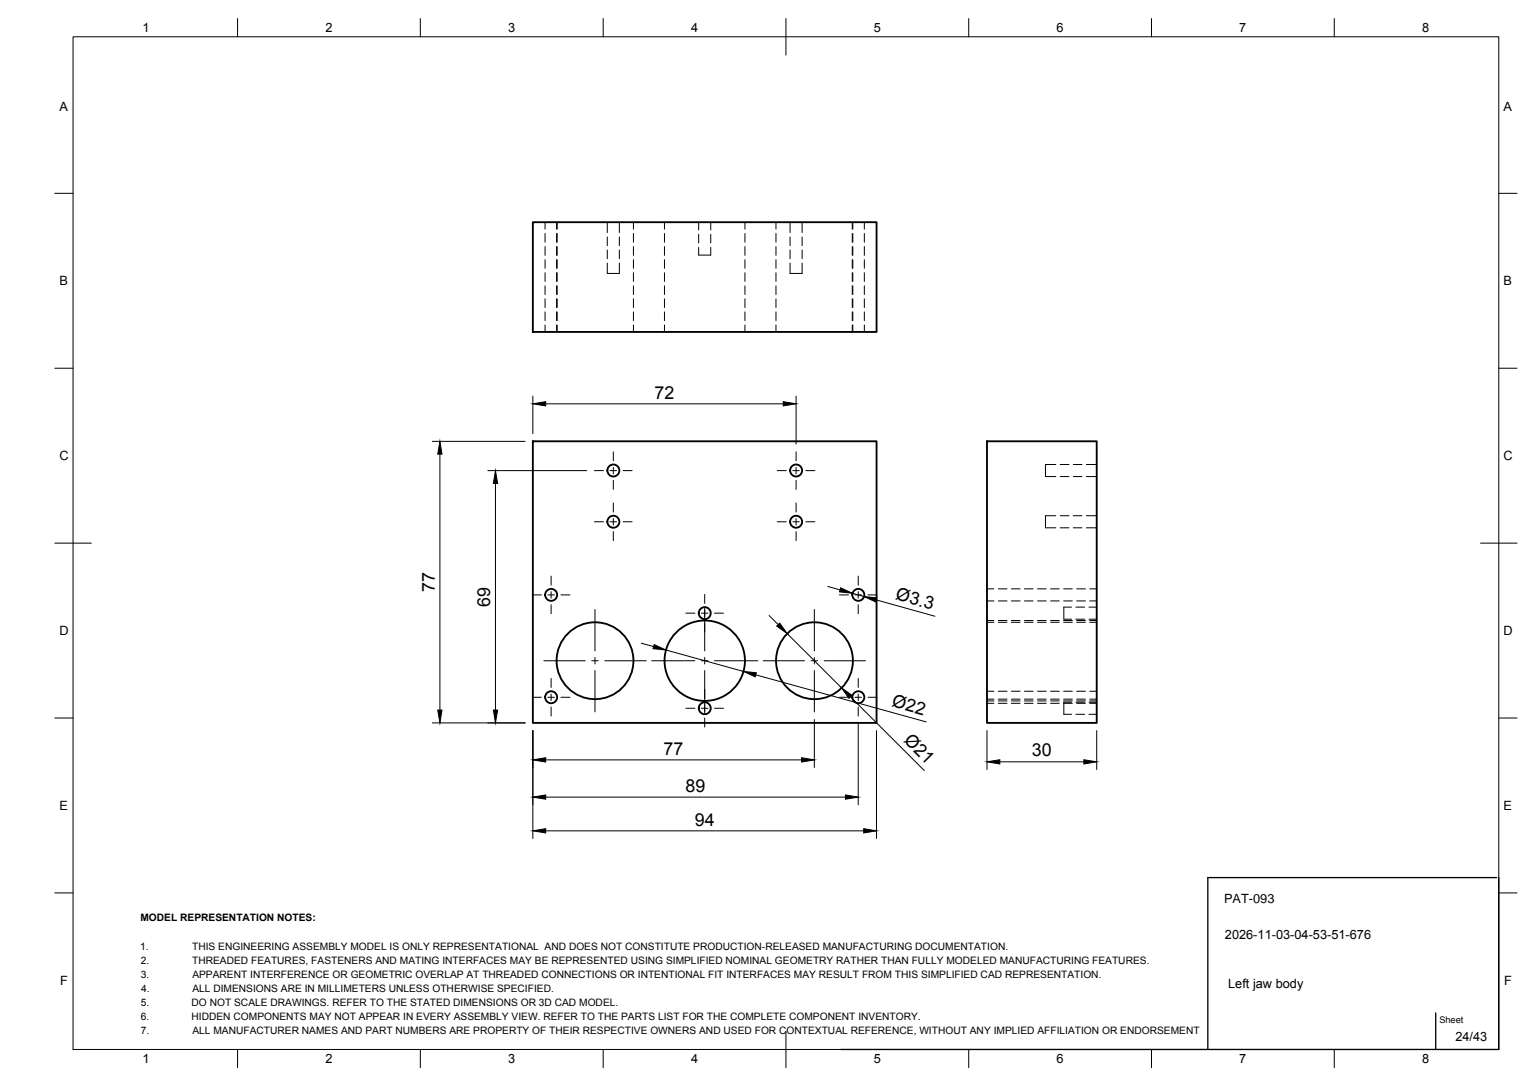
ISO-10303-21;
HEADER;
/* Generated by software containing ST-Developer
 * from STEP Tools, Inc. (www.steptools.com) 
 */

FILE_DESCRIPTION(
/* description */ ('Self-centering screw clamp'),
/* implementation_level */ '2;1');

FILE_NAME(
/* name */ 'Left jaw body.step',
/* time_stamp */ '2026-10-28T03:25:31-07:00',
/* author */ (''),
/* organization */ (''),
/* preprocessor_version */ 'ST-DEVELOPER v20.2',
/* originating_system */ 'Autodesk Translation Framework v15.17.0.0',
/* authorisation */ '');

FILE_SCHEMA (('AUTOMOTIVE_DESIGN { 1 0 10303 214 3 1 1 }'));
ENDSEC;

DATA;
#10=MECHANICAL_DESIGN_GEOMETRIC_PRESENTATION_REPRESENTATION('',(#650),#16799);
#561=SHAPE_REPRESENTATION_RELATIONSHIP('SRR','None',#17036,#602);
#602=ADVANCED_BREP_SHAPE_REPRESENTATION('',(#698),#16774);
#650=STYLED_ITEM('',(#17305),#698);
#698=MANIFOLD_SOLID_BREP('Body1',#9101);
#851=FACE_BOUND('',#2160,.T.);
#852=FACE_BOUND('',#2161,.T.);
#853=FACE_BOUND('',#2162,.T.);
#854=FACE_BOUND('',#2163,.T.);
#855=FACE_BOUND('',#2164,.T.);
#856=FACE_BOUND('',#2165,.T.);
#857=FACE_BOUND('',#2166,.T.);
#858=FACE_BOUND('',#2167,.T.);
#859=FACE_BOUND('',#2168,.T.);
#860=FACE_BOUND('',#2169,.T.);
#861=FACE_BOUND('',#2170,.T.);
#862=FACE_BOUND('',#2171,.T.);
#863=FACE_BOUND('',#2172,.T.);
#864=FACE_BOUND('',#2175,.T.);
#865=FACE_BOUND('',#2176,.T.);
#866=FACE_BOUND('',#2177,.T.);
#867=FACE_BOUND('',#2178,.T.);
#868=FACE_BOUND('',#2179,.T.);
#869=FACE_BOUND('',#2180,.T.);
#870=FACE_BOUND('',#2181,.T.);
#1122=PLANE('',#10087);
#1123=PLANE('',#10091);
#1124=PLANE('',#10095);
#1125=PLANE('',#10099);
#1126=PLANE('',#10103);
#1127=PLANE('',#10107);
#1128=PLANE('',#10129);
#1129=PLANE('',#10130);
#1130=PLANE('',#10131);
#1131=PLANE('',#10132);
#1132=PLANE('',#10133);
#1133=PLANE('',#10134);
#1502=FACE_OUTER_BOUND('',#2139,.T.);
#1503=FACE_OUTER_BOUND('',#2140,.T.);
#1504=FACE_OUTER_BOUND('',#2141,.T.);
#1505=FACE_OUTER_BOUND('',#2142,.T.);
#1506=FACE_OUTER_BOUND('',#2143,.T.);
#1507=FACE_OUTER_BOUND('',#2144,.T.);
#1508=FACE_OUTER_BOUND('',#2145,.T.);
#1509=FACE_OUTER_BOUND('',#2146,.T.);
#1510=FACE_OUTER_BOUND('',#2147,.T.);
#1511=FACE_OUTER_BOUND('',#2148,.T.);
#1512=FACE_OUTER_BOUND('',#2149,.T.);
#1513=FACE_OUTER_BOUND('',#2150,.T.);
#1514=FACE_OUTER_BOUND('',#2151,.T.);
#1515=FACE_OUTER_BOUND('',#2152,.T.);
#1516=FACE_OUTER_BOUND('',#2153,.T.);
#1517=FACE_OUTER_BOUND('',#2154,.T.);
#1518=FACE_OUTER_BOUND('',#2155,.T.);
#1519=FACE_OUTER_BOUND('',#2156,.T.);
#1520=FACE_OUTER_BOUND('',#2157,.T.);
#1521=FACE_OUTER_BOUND('',#2158,.T.);
#1522=FACE_OUTER_BOUND('',#2159,.T.);
#1523=FACE_OUTER_BOUND('',#2173,.T.);
#1524=FACE_OUTER_BOUND('',#2174,.T.);
#1525=FACE_OUTER_BOUND('',#2182,.T.);
#1526=FACE_OUTER_BOUND('',#2183,.T.);
#2139=EDGE_LOOP('',(#7191,#7192,#7193,#7194));
#2140=EDGE_LOOP('',(#7195));
#2141=EDGE_LOOP('',(#7196,#7197,#7198,#7199));
#2142=EDGE_LOOP('',(#7200));
#2143=EDGE_LOOP('',(#7201,#7202,#7203,#7204));
#2144=EDGE_LOOP('',(#7205));
#2145=EDGE_LOOP('',(#7206,#7207,#7208,#7209));
#2146=EDGE_LOOP('',(#7210));
#2147=EDGE_LOOP('',(#7211,#7212,#7213,#7214));
#2148=EDGE_LOOP('',(#7215));
#2149=EDGE_LOOP('',(#7216,#7217,#7218,#7219));
#2150=EDGE_LOOP('',(#7220));
#2151=EDGE_LOOP('',(#7221,#7222,#7223,#7224));
#2152=EDGE_LOOP('',(#7225,#7226,#7227,#7228));
#2153=EDGE_LOOP('',(#7229,#7230,#7231,#7232));
#2154=EDGE_LOOP('',(#7233,#7234,#7235,#7236));
#2155=EDGE_LOOP('',(#7237,#7238,#7239,#7240));
#2156=EDGE_LOOP('',(#7241,#7242,#7243,#7244));
#2157=EDGE_LOOP('',(#7245,#7246,#7247,#7248));
#2158=EDGE_LOOP('',(#7249,#7250,#7251,#7252));
#2159=EDGE_LOOP('',(#7253,#7254,#7255,#7256));
#2160=EDGE_LOOP('',(#7257));
#2161=EDGE_LOOP('',(#7258));
#2162=EDGE_LOOP('',(#7259));
#2163=EDGE_LOOP('',(#7260));
#2164=EDGE_LOOP('',(#7261));
#2165=EDGE_LOOP('',(#7262));
#2166=EDGE_LOOP('',(#7263));
#2167=EDGE_LOOP('',(#7264));
#2168=EDGE_LOOP('',(#7265));
#2169=EDGE_LOOP('',(#7266));
#2170=EDGE_LOOP('',(#7267));
#2171=EDGE_LOOP('',(#7268));
#2172=EDGE_LOOP('',(#7269));
#2173=EDGE_LOOP('',(#7270,#7271,#7272,#7273));
#2174=EDGE_LOOP('',(#7274,#7275,#7276,#7277));
#2175=EDGE_LOOP('',(#7278));
#2176=EDGE_LOOP('',(#7279));
#2177=EDGE_LOOP('',(#7280));
#2178=EDGE_LOOP('',(#7281));
#2179=EDGE_LOOP('',(#7282));
#2180=EDGE_LOOP('',(#7283));
#2181=EDGE_LOOP('',(#7284));
#2182=EDGE_LOOP('',(#7285,#7286,#7287,#7288));
#2183=EDGE_LOOP('',(#7289,#7290,#7291,#7292));
#2842=LINE('',#15213,#3415);
#2843=LINE('',#15220,#3416);
#2844=LINE('',#15227,#3417);
#2845=LINE('',#15234,#3418);
#2846=LINE('',#15241,#3419);
#2847=LINE('',#15248,#3420);
#2848=LINE('',#15255,#3421);
#2849=LINE('',#15261,#3422);
#2850=LINE('',#15267,#3423);
#2851=LINE('',#15273,#3424);
#2852=LINE('',#15279,#3425);
#2853=LINE('',#15285,#3426);
#2854=LINE('',#15291,#3427);
#2855=LINE('',#15296,#3428);
#2856=LINE('',#15298,#3429);
#2857=LINE('',#15300,#3430);
#2858=LINE('',#15301,#3431);
#2859=LINE('',#15304,#3432);
#2860=LINE('',#15306,#3433);
#2861=LINE('',#15307,#3434);
#2862=LINE('',#15310,#3435);
#2863=LINE('',#15312,#3436);
#2864=LINE('',#15313,#3437);
#2865=LINE('',#15315,#3438);
#2866=LINE('',#15316,#3439);
#3415=VECTOR('',#12035,0.165);
#3416=VECTOR('',#12044,0.164999999999999);
#3417=VECTOR('',#12053,0.165);
#3418=VECTOR('',#12062,0.164999999999999);
#3419=VECTOR('',#12071,0.165);
#3420=VECTOR('',#12080,0.165);
#3421=VECTOR('',#12089,0.165);
#3422=VECTOR('',#12096,0.165);
#3423=VECTOR('',#12103,0.165);
#3424=VECTOR('',#12110,0.165);
#3425=VECTOR('',#12117,1.1);
#3426=VECTOR('',#12124,1.05);
#3427=VECTOR('',#12131,1.05);
#3428=VECTOR('',#12136,1.);
#3429=VECTOR('',#12137,1.);
#3430=VECTOR('',#12138,1.);
#3431=VECTOR('',#12139,1.);
#3432=VECTOR('',#12142,1.);
#3433=VECTOR('',#12143,1.);
#3434=VECTOR('',#12144,1.);
#3435=VECTOR('',#12147,1.);
#3436=VECTOR('',#12148,1.);
#3437=VECTOR('',#12149,1.);
#3438=VECTOR('',#12152,1.);
#3439=VECTOR('',#12153,1.);
#3972=CIRCLE('',#10085,0.165);
#3973=CIRCLE('',#10086,0.165);
#3974=CIRCLE('',#10089,0.164999999999999);
#3975=CIRCLE('',#10090,0.164999999999999);
#3976=CIRCLE('',#10093,0.165);
#3977=CIRCLE('',#10094,0.165);
#3978=CIRCLE('',#10097,0.164999999999999);
#3979=CIRCLE('',#10098,0.164999999999999);
#3980=CIRCLE('',#10101,0.165);
#3981=CIRCLE('',#10102,0.165);
#3982=CIRCLE('',#10105,0.165);
#3983=CIRCLE('',#10106,0.165);
#3984=CIRCLE('',#10109,0.165);
#3985=CIRCLE('',#10110,0.165);
#3986=CIRCLE('',#10112,0.165);
#3987=CIRCLE('',#10113,0.165);
#3988=CIRCLE('',#10115,0.165);
#3989=CIRCLE('',#10116,0.165);
#3990=CIRCLE('',#10118,0.165);
#3991=CIRCLE('',#10119,0.165);
#3992=CIRCLE('',#10121,1.1);
#3993=CIRCLE('',#10122,1.1);
#3994=CIRCLE('',#10124,1.05);
#3995=CIRCLE('',#10125,1.05);
#3996=CIRCLE('',#10127,1.05);
#3997=CIRCLE('',#10128,1.05);
#4591=VERTEX_POINT('',#15210);
#4592=VERTEX_POINT('',#15212);
#4593=VERTEX_POINT('',#15217);
#4594=VERTEX_POINT('',#15219);
#4595=VERTEX_POINT('',#15224);
#4596=VERTEX_POINT('',#15226);
#4597=VERTEX_POINT('',#15231);
#4598=VERTEX_POINT('',#15233);
#4599=VERTEX_POINT('',#15238);
#4600=VERTEX_POINT('',#15240);
#4601=VERTEX_POINT('',#15245);
#4602=VERTEX_POINT('',#15247);
#4603=VERTEX_POINT('',#15252);
#4604=VERTEX_POINT('',#15254);
#4605=VERTEX_POINT('',#15258);
#4606=VERTEX_POINT('',#15260);
#4607=VERTEX_POINT('',#15264);
#4608=VERTEX_POINT('',#15266);
#4609=VERTEX_POINT('',#15270);
#4610=VERTEX_POINT('',#15272);
#4611=VERTEX_POINT('',#15276);
#4612=VERTEX_POINT('',#15278);
#4613=VERTEX_POINT('',#15282);
#4614=VERTEX_POINT('',#15284);
#4615=VERTEX_POINT('',#15288);
#4616=VERTEX_POINT('',#15290);
#4617=VERTEX_POINT('',#15294);
#4618=VERTEX_POINT('',#15295);
#4619=VERTEX_POINT('',#15297);
#4620=VERTEX_POINT('',#15299);
#4621=VERTEX_POINT('',#15303);
#4622=VERTEX_POINT('',#15305);
#4623=VERTEX_POINT('',#15309);
#4624=VERTEX_POINT('',#15311);
#5520=EDGE_CURVE('',#4591,#4591,#3972,.T.);
#5521=EDGE_CURVE('',#4591,#4592,#2842,.T.);
#5522=EDGE_CURVE('',#4592,#4592,#3973,.T.);
#5523=EDGE_CURVE('',#4593,#4593,#3974,.T.);
#5524=EDGE_CURVE('',#4593,#4594,#2843,.T.);
#5525=EDGE_CURVE('',#4594,#4594,#3975,.T.);
#5526=EDGE_CURVE('',#4595,#4595,#3976,.T.);
#5527=EDGE_CURVE('',#4595,#4596,#2844,.T.);
#5528=EDGE_CURVE('',#4596,#4596,#3977,.T.);
#5529=EDGE_CURVE('',#4597,#4597,#3978,.T.);
#5530=EDGE_CURVE('',#4597,#4598,#2845,.T.);
#5531=EDGE_CURVE('',#4598,#4598,#3979,.T.);
#5532=EDGE_CURVE('',#4599,#4599,#3980,.T.);
#5533=EDGE_CURVE('',#4599,#4600,#2846,.T.);
#5534=EDGE_CURVE('',#4600,#4600,#3981,.T.);
#5535=EDGE_CURVE('',#4601,#4601,#3982,.T.);
#5536=EDGE_CURVE('',#4601,#4602,#2847,.T.);
#5537=EDGE_CURVE('',#4602,#4602,#3983,.T.);
#5538=EDGE_CURVE('',#4603,#4603,#3984,.T.);
#5539=EDGE_CURVE('',#4603,#4604,#2848,.T.);
#5540=EDGE_CURVE('',#4604,#4604,#3985,.T.);
#5541=EDGE_CURVE('',#4605,#4605,#3986,.T.);
#5542=EDGE_CURVE('',#4605,#4606,#2849,.T.);
#5543=EDGE_CURVE('',#4606,#4606,#3987,.T.);
#5544=EDGE_CURVE('',#4607,#4607,#3988,.T.);
#5545=EDGE_CURVE('',#4607,#4608,#2850,.T.);
#5546=EDGE_CURVE('',#4608,#4608,#3989,.T.);
#5547=EDGE_CURVE('',#4609,#4609,#3990,.T.);
#5548=EDGE_CURVE('',#4609,#4610,#2851,.T.);
#5549=EDGE_CURVE('',#4610,#4610,#3991,.T.);
#5550=EDGE_CURVE('',#4611,#4611,#3992,.T.);
#5551=EDGE_CURVE('',#4611,#4612,#2852,.T.);
#5552=EDGE_CURVE('',#4612,#4612,#3993,.T.);
#5553=EDGE_CURVE('',#4613,#4613,#3994,.T.);
#5554=EDGE_CURVE('',#4613,#4614,#2853,.T.);
#5555=EDGE_CURVE('',#4614,#4614,#3995,.T.);
#5556=EDGE_CURVE('',#4615,#4615,#3996,.T.);
#5557=EDGE_CURVE('',#4615,#4616,#2854,.T.);
#5558=EDGE_CURVE('',#4616,#4616,#3997,.T.);
#5559=EDGE_CURVE('',#4617,#4618,#2855,.T.);
#5560=EDGE_CURVE('',#4618,#4619,#2856,.T.);
#5561=EDGE_CURVE('',#4620,#4619,#2857,.T.);
#5562=EDGE_CURVE('',#4617,#4620,#2858,.T.);
#5563=EDGE_CURVE('',#4621,#4617,#2859,.T.);
#5564=EDGE_CURVE('',#4622,#4620,#2860,.T.);
#5565=EDGE_CURVE('',#4621,#4622,#2861,.T.);
#5566=EDGE_CURVE('',#4623,#4621,#2862,.T.);
#5567=EDGE_CURVE('',#4624,#4622,#2863,.T.);
#5568=EDGE_CURVE('',#4623,#4624,#2864,.T.);
#5569=EDGE_CURVE('',#4618,#4623,#2865,.T.);
#5570=EDGE_CURVE('',#4619,#4624,#2866,.T.);
#7191=ORIENTED_EDGE('',*,*,#5520,.F.);
#7192=ORIENTED_EDGE('',*,*,#5521,.T.);
#7193=ORIENTED_EDGE('',*,*,#5522,.F.);
#7194=ORIENTED_EDGE('',*,*,#5521,.F.);
#7195=ORIENTED_EDGE('',*,*,#5520,.T.);
#7196=ORIENTED_EDGE('',*,*,#5523,.F.);
#7197=ORIENTED_EDGE('',*,*,#5524,.T.);
#7198=ORIENTED_EDGE('',*,*,#5525,.F.);
#7199=ORIENTED_EDGE('',*,*,#5524,.F.);
#7200=ORIENTED_EDGE('',*,*,#5523,.T.);
#7201=ORIENTED_EDGE('',*,*,#5526,.F.);
#7202=ORIENTED_EDGE('',*,*,#5527,.T.);
#7203=ORIENTED_EDGE('',*,*,#5528,.F.);
#7204=ORIENTED_EDGE('',*,*,#5527,.F.);
#7205=ORIENTED_EDGE('',*,*,#5526,.T.);
#7206=ORIENTED_EDGE('',*,*,#5529,.F.);
#7207=ORIENTED_EDGE('',*,*,#5530,.T.);
#7208=ORIENTED_EDGE('',*,*,#5531,.F.);
#7209=ORIENTED_EDGE('',*,*,#5530,.F.);
#7210=ORIENTED_EDGE('',*,*,#5529,.T.);
#7211=ORIENTED_EDGE('',*,*,#5532,.F.);
#7212=ORIENTED_EDGE('',*,*,#5533,.T.);
#7213=ORIENTED_EDGE('',*,*,#5534,.F.);
#7214=ORIENTED_EDGE('',*,*,#5533,.F.);
#7215=ORIENTED_EDGE('',*,*,#5532,.T.);
#7216=ORIENTED_EDGE('',*,*,#5535,.F.);
#7217=ORIENTED_EDGE('',*,*,#5536,.T.);
#7218=ORIENTED_EDGE('',*,*,#5537,.F.);
#7219=ORIENTED_EDGE('',*,*,#5536,.F.);
#7220=ORIENTED_EDGE('',*,*,#5535,.T.);
#7221=ORIENTED_EDGE('',*,*,#5538,.F.);
#7222=ORIENTED_EDGE('',*,*,#5539,.T.);
#7223=ORIENTED_EDGE('',*,*,#5540,.F.);
#7224=ORIENTED_EDGE('',*,*,#5539,.F.);
#7225=ORIENTED_EDGE('',*,*,#5541,.F.);
#7226=ORIENTED_EDGE('',*,*,#5542,.T.);
#7227=ORIENTED_EDGE('',*,*,#5543,.F.);
#7228=ORIENTED_EDGE('',*,*,#5542,.F.);
#7229=ORIENTED_EDGE('',*,*,#5544,.F.);
#7230=ORIENTED_EDGE('',*,*,#5545,.T.);
#7231=ORIENTED_EDGE('',*,*,#5546,.F.);
#7232=ORIENTED_EDGE('',*,*,#5545,.F.);
#7233=ORIENTED_EDGE('',*,*,#5547,.F.);
#7234=ORIENTED_EDGE('',*,*,#5548,.T.);
#7235=ORIENTED_EDGE('',*,*,#5549,.F.);
#7236=ORIENTED_EDGE('',*,*,#5548,.F.);
#7237=ORIENTED_EDGE('',*,*,#5550,.F.);
#7238=ORIENTED_EDGE('',*,*,#5551,.T.);
#7239=ORIENTED_EDGE('',*,*,#5552,.F.);
#7240=ORIENTED_EDGE('',*,*,#5551,.F.);
#7241=ORIENTED_EDGE('',*,*,#5553,.F.);
#7242=ORIENTED_EDGE('',*,*,#5554,.T.);
#7243=ORIENTED_EDGE('',*,*,#5555,.F.);
#7244=ORIENTED_EDGE('',*,*,#5554,.F.);
#7245=ORIENTED_EDGE('',*,*,#5556,.F.);
#7246=ORIENTED_EDGE('',*,*,#5557,.T.);
#7247=ORIENTED_EDGE('',*,*,#5558,.F.);
#7248=ORIENTED_EDGE('',*,*,#5557,.F.);
#7249=ORIENTED_EDGE('',*,*,#5559,.T.);
#7250=ORIENTED_EDGE('',*,*,#5560,.T.);
#7251=ORIENTED_EDGE('',*,*,#5561,.F.);
#7252=ORIENTED_EDGE('',*,*,#5562,.F.);
#7253=ORIENTED_EDGE('',*,*,#5563,.T.);
#7254=ORIENTED_EDGE('',*,*,#5562,.T.);
#7255=ORIENTED_EDGE('',*,*,#5564,.F.);
#7256=ORIENTED_EDGE('',*,*,#5565,.F.);
#7257=ORIENTED_EDGE('',*,*,#5534,.T.);
#7258=ORIENTED_EDGE('',*,*,#5537,.T.);
#7259=ORIENTED_EDGE('',*,*,#5558,.T.);
#7260=ORIENTED_EDGE('',*,*,#5555,.T.);
#7261=ORIENTED_EDGE('',*,*,#5552,.T.);
#7262=ORIENTED_EDGE('',*,*,#5549,.T.);
#7263=ORIENTED_EDGE('',*,*,#5546,.T.);
#7264=ORIENTED_EDGE('',*,*,#5543,.T.);
#7265=ORIENTED_EDGE('',*,*,#5540,.T.);
#7266=ORIENTED_EDGE('',*,*,#5531,.T.);
#7267=ORIENTED_EDGE('',*,*,#5528,.T.);
#7268=ORIENTED_EDGE('',*,*,#5525,.T.);
#7269=ORIENTED_EDGE('',*,*,#5522,.T.);
#7270=ORIENTED_EDGE('',*,*,#5566,.T.);
#7271=ORIENTED_EDGE('',*,*,#5565,.T.);
#7272=ORIENTED_EDGE('',*,*,#5567,.F.);
#7273=ORIENTED_EDGE('',*,*,#5568,.F.);
#7274=ORIENTED_EDGE('',*,*,#5569,.T.);
#7275=ORIENTED_EDGE('',*,*,#5568,.T.);
#7276=ORIENTED_EDGE('',*,*,#5570,.F.);
#7277=ORIENTED_EDGE('',*,*,#5560,.F.);
#7278=ORIENTED_EDGE('',*,*,#5556,.T.);
#7279=ORIENTED_EDGE('',*,*,#5553,.T.);
#7280=ORIENTED_EDGE('',*,*,#5550,.T.);
#7281=ORIENTED_EDGE('',*,*,#5547,.T.);
#7282=ORIENTED_EDGE('',*,*,#5544,.T.);
#7283=ORIENTED_EDGE('',*,*,#5541,.T.);
#7284=ORIENTED_EDGE('',*,*,#5538,.T.);
#7285=ORIENTED_EDGE('',*,*,#5570,.T.);
#7286=ORIENTED_EDGE('',*,*,#5567,.T.);
#7287=ORIENTED_EDGE('',*,*,#5564,.T.);
#7288=ORIENTED_EDGE('',*,*,#5561,.T.);
#7289=ORIENTED_EDGE('',*,*,#5569,.F.);
#7290=ORIENTED_EDGE('',*,*,#5559,.F.);
#7291=ORIENTED_EDGE('',*,*,#5563,.F.);
#7292=ORIENTED_EDGE('',*,*,#5566,.F.);
#8456=CYLINDRICAL_SURFACE('',#10084,0.165);
#8457=CYLINDRICAL_SURFACE('',#10088,0.164999999999999);
#8458=CYLINDRICAL_SURFACE('',#10092,0.165);
#8459=CYLINDRICAL_SURFACE('',#10096,0.164999999999999);
#8460=CYLINDRICAL_SURFACE('',#10100,0.165);
#8461=CYLINDRICAL_SURFACE('',#10104,0.165);
#8462=CYLINDRICAL_SURFACE('',#10108,0.165);
#8463=CYLINDRICAL_SURFACE('',#10111,0.165);
#8464=CYLINDRICAL_SURFACE('',#10114,0.165);
#8465=CYLINDRICAL_SURFACE('',#10117,0.165);
#8466=CYLINDRICAL_SURFACE('',#10120,1.1);
#8467=CYLINDRICAL_SURFACE('',#10123,1.05);
#8468=CYLINDRICAL_SURFACE('',#10126,1.05);
#8800=ADVANCED_FACE('',(#1502),#8456,.F.);
#8801=ADVANCED_FACE('',(#1503),#1122,.T.);
#8802=ADVANCED_FACE('',(#1504),#8457,.F.);
#8803=ADVANCED_FACE('',(#1505),#1123,.T.);
#8804=ADVANCED_FACE('',(#1506),#8458,.F.);
#8805=ADVANCED_FACE('',(#1507),#1124,.T.);
#8806=ADVANCED_FACE('',(#1508),#8459,.F.);
#8807=ADVANCED_FACE('',(#1509),#1125,.T.);
#8808=ADVANCED_FACE('',(#1510),#8460,.F.);
#8809=ADVANCED_FACE('',(#1511),#1126,.T.);
#8810=ADVANCED_FACE('',(#1512),#8461,.F.);
#8811=ADVANCED_FACE('',(#1513),#1127,.T.);
#8812=ADVANCED_FACE('',(#1514),#8462,.F.);
#8813=ADVANCED_FACE('',(#1515),#8463,.F.);
#8814=ADVANCED_FACE('',(#1516),#8464,.F.);
#8815=ADVANCED_FACE('',(#1517),#8465,.F.);
#8816=ADVANCED_FACE('',(#1518),#8466,.F.);
#8817=ADVANCED_FACE('',(#1519),#8467,.F.);
#8818=ADVANCED_FACE('',(#1520),#8468,.F.);
#8819=ADVANCED_FACE('',(#1521),#1128,.T.);
#8820=ADVANCED_FACE('',(#1522,#851,#852,#853,#854,#855,#856,#857,#858,#859,
#860,#861,#862,#863),#1129,.T.);
#8821=ADVANCED_FACE('',(#1523),#1130,.T.);
#8822=ADVANCED_FACE('',(#1524,#864,#865,#866,#867,#868,#869,#870),#1131,
 .T.);
#8823=ADVANCED_FACE('',(#1525),#1132,.T.);
#8824=ADVANCED_FACE('',(#1526),#1133,.F.);
#9101=CLOSED_SHELL('',(#8800,#8801,#8802,#8803,#8804,#8805,#8806,#8807,
#8808,#8809,#8810,#8811,#8812,#8813,#8814,#8815,#8816,#8817,#8818,#8819,
#8820,#8821,#8822,#8823,#8824));
#10083=AXIS2_PLACEMENT_3D('',#15208,#12029,#12030);
#10084=AXIS2_PLACEMENT_3D('',#15209,#12031,#12032);
#10085=AXIS2_PLACEMENT_3D('',#15211,#12033,#12034);
#10086=AXIS2_PLACEMENT_3D('',#15214,#12036,#12037);
#10087=AXIS2_PLACEMENT_3D('',#15215,#12038,#12039);
#10088=AXIS2_PLACEMENT_3D('',#15216,#12040,#12041);
#10089=AXIS2_PLACEMENT_3D('',#15218,#12042,#12043);
#10090=AXIS2_PLACEMENT_3D('',#15221,#12045,#12046);
#10091=AXIS2_PLACEMENT_3D('',#15222,#12047,#12048);
#10092=AXIS2_PLACEMENT_3D('',#15223,#12049,#12050);
#10093=AXIS2_PLACEMENT_3D('',#15225,#12051,#12052);
#10094=AXIS2_PLACEMENT_3D('',#15228,#12054,#12055);
#10095=AXIS2_PLACEMENT_3D('',#15229,#12056,#12057);
#10096=AXIS2_PLACEMENT_3D('',#15230,#12058,#12059);
#10097=AXIS2_PLACEMENT_3D('',#15232,#12060,#12061);
#10098=AXIS2_PLACEMENT_3D('',#15235,#12063,#12064);
#10099=AXIS2_PLACEMENT_3D('',#15236,#12065,#12066);
#10100=AXIS2_PLACEMENT_3D('',#15237,#12067,#12068);
#10101=AXIS2_PLACEMENT_3D('',#15239,#12069,#12070);
#10102=AXIS2_PLACEMENT_3D('',#15242,#12072,#12073);
#10103=AXIS2_PLACEMENT_3D('',#15243,#12074,#12075);
#10104=AXIS2_PLACEMENT_3D('',#15244,#12076,#12077);
#10105=AXIS2_PLACEMENT_3D('',#15246,#12078,#12079);
#10106=AXIS2_PLACEMENT_3D('',#15249,#12081,#12082);
#10107=AXIS2_PLACEMENT_3D('',#15250,#12083,#12084);
#10108=AXIS2_PLACEMENT_3D('',#15251,#12085,#12086);
#10109=AXIS2_PLACEMENT_3D('',#15253,#12087,#12088);
#10110=AXIS2_PLACEMENT_3D('',#15256,#12090,#12091);
#10111=AXIS2_PLACEMENT_3D('',#15257,#12092,#12093);
#10112=AXIS2_PLACEMENT_3D('',#15259,#12094,#12095);
#10113=AXIS2_PLACEMENT_3D('',#15262,#12097,#12098);
#10114=AXIS2_PLACEMENT_3D('',#15263,#12099,#12100);
#10115=AXIS2_PLACEMENT_3D('',#15265,#12101,#12102);
#10116=AXIS2_PLACEMENT_3D('',#15268,#12104,#12105);
#10117=AXIS2_PLACEMENT_3D('',#15269,#12106,#12107);
#10118=AXIS2_PLACEMENT_3D('',#15271,#12108,#12109);
#10119=AXIS2_PLACEMENT_3D('',#15274,#12111,#12112);
#10120=AXIS2_PLACEMENT_3D('',#15275,#12113,#12114);
#10121=AXIS2_PLACEMENT_3D('',#15277,#12115,#12116);
#10122=AXIS2_PLACEMENT_3D('',#15280,#12118,#12119);
#10123=AXIS2_PLACEMENT_3D('',#15281,#12120,#12121);
#10124=AXIS2_PLACEMENT_3D('',#15283,#12122,#12123);
#10125=AXIS2_PLACEMENT_3D('',#15286,#12125,#12126);
#10126=AXIS2_PLACEMENT_3D('',#15287,#12127,#12128);
#10127=AXIS2_PLACEMENT_3D('',#15289,#12129,#12130);
#10128=AXIS2_PLACEMENT_3D('',#15292,#12132,#12133);
#10129=AXIS2_PLACEMENT_3D('',#15293,#12134,#12135);
#10130=AXIS2_PLACEMENT_3D('',#15302,#12140,#12141);
#10131=AXIS2_PLACEMENT_3D('',#15308,#12145,#12146);
#10132=AXIS2_PLACEMENT_3D('',#15314,#12150,#12151);
#10133=AXIS2_PLACEMENT_3D('',#15317,#12154,#12155);
#10134=AXIS2_PLACEMENT_3D('',#15318,#12156,#12157);
#12029=DIRECTION('axis',(0.,0.,1.));
#12030=DIRECTION('refdir',(1.,0.,0.));
#12031=DIRECTION('center_axis',(1.,0.,0.));
#12032=DIRECTION('ref_axis',(0.,0.,-1.));
#12033=DIRECTION('center_axis',(1.,0.,0.));
#12034=DIRECTION('ref_axis',(0.,0.,-1.));
#12035=DIRECTION('',(1.,0.,0.));
#12036=DIRECTION('center_axis',(-1.,0.,0.));
#12037=DIRECTION('ref_axis',(0.,0.,-1.));
#12038=DIRECTION('center_axis',(1.,0.,0.));
#12039=DIRECTION('ref_axis',(0.,0.,-1.));
#12040=DIRECTION('center_axis',(1.,0.,0.));
#12041=DIRECTION('ref_axis',(0.,0.,-1.));
#12042=DIRECTION('center_axis',(1.,0.,0.));
#12043=DIRECTION('ref_axis',(0.,0.,-1.));
#12044=DIRECTION('',(1.,0.,0.));
#12045=DIRECTION('center_axis',(-1.,0.,0.));
#12046=DIRECTION('ref_axis',(0.,0.,-1.));
#12047=DIRECTION('center_axis',(1.,0.,0.));
#12048=DIRECTION('ref_axis',(0.,0.,-1.));
#12049=DIRECTION('center_axis',(1.,0.,0.));
#12050=DIRECTION('ref_axis',(0.,0.,-1.));
#12051=DIRECTION('center_axis',(1.,0.,0.));
#12052=DIRECTION('ref_axis',(0.,0.,-1.));
#12053=DIRECTION('',(1.,0.,0.));
#12054=DIRECTION('center_axis',(-1.,0.,0.));
#12055=DIRECTION('ref_axis',(0.,0.,-1.));
#12056=DIRECTION('center_axis',(1.,0.,0.));
#12057=DIRECTION('ref_axis',(0.,0.,-1.));
#12058=DIRECTION('center_axis',(1.,0.,0.));
#12059=DIRECTION('ref_axis',(0.,0.,-1.));
#12060=DIRECTION('center_axis',(1.,0.,0.));
#12061=DIRECTION('ref_axis',(0.,0.,-1.));
#12062=DIRECTION('',(1.,0.,0.));
#12063=DIRECTION('center_axis',(-1.,0.,0.));
#12064=DIRECTION('ref_axis',(0.,0.,-1.));
#12065=DIRECTION('center_axis',(1.,0.,0.));
#12066=DIRECTION('ref_axis',(0.,0.,-1.));
#12067=DIRECTION('center_axis',(1.,0.,0.));
#12068=DIRECTION('ref_axis',(0.,0.,-1.));
#12069=DIRECTION('center_axis',(1.,0.,0.));
#12070=DIRECTION('ref_axis',(0.,0.,-1.));
#12071=DIRECTION('',(1.,0.,0.));
#12072=DIRECTION('center_axis',(-1.,0.,0.));
#12073=DIRECTION('ref_axis',(0.,0.,-1.));
#12074=DIRECTION('center_axis',(1.,0.,0.));
#12075=DIRECTION('ref_axis',(0.,0.,-1.));
#12076=DIRECTION('center_axis',(1.,0.,0.));
#12077=DIRECTION('ref_axis',(0.,0.,-1.));
#12078=DIRECTION('center_axis',(1.,0.,0.));
#12079=DIRECTION('ref_axis',(0.,0.,-1.));
#12080=DIRECTION('',(1.,0.,0.));
#12081=DIRECTION('center_axis',(-1.,0.,0.));
#12082=DIRECTION('ref_axis',(0.,0.,-1.));
#12083=DIRECTION('center_axis',(1.,0.,0.));
#12084=DIRECTION('ref_axis',(0.,0.,-1.));
#12085=DIRECTION('center_axis',(1.,0.,0.));
#12086=DIRECTION('ref_axis',(0.,0.,-1.));
#12087=DIRECTION('center_axis',(1.,0.,0.));
#12088=DIRECTION('ref_axis',(0.,0.,-1.));
#12089=DIRECTION('',(1.,0.,0.));
#12090=DIRECTION('center_axis',(-1.,0.,0.));
#12091=DIRECTION('ref_axis',(0.,0.,-1.));
#12092=DIRECTION('center_axis',(1.,0.,0.));
#12093=DIRECTION('ref_axis',(0.,0.,-1.));
#12094=DIRECTION('center_axis',(1.,0.,0.));
#12095=DIRECTION('ref_axis',(0.,0.,-1.));
#12096=DIRECTION('',(1.,0.,0.));
#12097=DIRECTION('center_axis',(-1.,0.,0.));
#12098=DIRECTION('ref_axis',(0.,0.,-1.));
#12099=DIRECTION('center_axis',(1.,0.,0.));
#12100=DIRECTION('ref_axis',(0.,0.,-1.));
#12101=DIRECTION('center_axis',(1.,0.,0.));
#12102=DIRECTION('ref_axis',(0.,0.,-1.));
#12103=DIRECTION('',(1.,0.,0.));
#12104=DIRECTION('center_axis',(-1.,0.,0.));
#12105=DIRECTION('ref_axis',(0.,0.,-1.));
#12106=DIRECTION('center_axis',(1.,0.,0.));
#12107=DIRECTION('ref_axis',(0.,0.,-1.));
#12108=DIRECTION('center_axis',(1.,0.,0.));
#12109=DIRECTION('ref_axis',(0.,0.,-1.));
#12110=DIRECTION('',(1.,0.,0.));
#12111=DIRECTION('center_axis',(-1.,0.,0.));
#12112=DIRECTION('ref_axis',(0.,0.,-1.));
#12113=DIRECTION('center_axis',(1.,0.,0.));
#12114=DIRECTION('ref_axis',(0.,0.,-1.));
#12115=DIRECTION('center_axis',(1.,0.,0.));
#12116=DIRECTION('ref_axis',(0.,0.,-1.));
#12117=DIRECTION('',(1.,0.,0.));
#12118=DIRECTION('center_axis',(-1.,0.,0.));
#12119=DIRECTION('ref_axis',(0.,0.,-1.));
#12120=DIRECTION('center_axis',(1.,0.,0.));
#12121=DIRECTION('ref_axis',(0.,0.,-1.));
#12122=DIRECTION('center_axis',(1.,0.,0.));
#12123=DIRECTION('ref_axis',(0.,0.,-1.));
#12124=DIRECTION('',(1.,0.,0.));
#12125=DIRECTION('center_axis',(-1.,0.,0.));
#12126=DIRECTION('ref_axis',(0.,0.,-1.));
#12127=DIRECTION('center_axis',(1.,0.,0.));
#12128=DIRECTION('ref_axis',(0.,0.,-1.));
#12129=DIRECTION('center_axis',(1.,0.,0.));
#12130=DIRECTION('ref_axis',(0.,0.,-1.));
#12131=DIRECTION('',(1.,0.,0.));
#12132=DIRECTION('center_axis',(-1.,0.,0.));
#12133=DIRECTION('ref_axis',(0.,0.,-1.));
#12134=DIRECTION('center_axis',(0.,1.,0.));
#12135=DIRECTION('ref_axis',(-1.,0.,0.));
#12136=DIRECTION('',(-1.,0.,0.));
#12137=DIRECTION('',(0.,0.,1.));
#12138=DIRECTION('',(-1.,0.,0.));
#12139=DIRECTION('',(0.,0.,1.));
#12140=DIRECTION('center_axis',(1.,0.,0.));
#12141=DIRECTION('ref_axis',(0.,1.,0.));
#12142=DIRECTION('',(0.,1.,0.));
#12143=DIRECTION('',(0.,1.,0.));
#12144=DIRECTION('',(0.,0.,1.));
#12145=DIRECTION('center_axis',(0.,-1.,0.));
#12146=DIRECTION('ref_axis',(1.,0.,0.));
#12147=DIRECTION('',(1.,0.,0.));
#12148=DIRECTION('',(1.,0.,0.));
#12149=DIRECTION('',(0.,0.,1.));
#12150=DIRECTION('center_axis',(-1.,0.,0.));
#12151=DIRECTION('ref_axis',(0.,-1.,0.));
#12152=DIRECTION('',(0.,-1.,0.));
#12153=DIRECTION('',(0.,-1.,0.));
#12154=DIRECTION('center_axis',(0.,0.,1.));
#12155=DIRECTION('ref_axis',(1.,0.,0.));
#12156=DIRECTION('center_axis',(0.,0.,1.));
#12157=DIRECTION('ref_axis',(1.,0.,0.));
#15208=CARTESIAN_POINT('',(0.,0.,0.));
#15209=CARTESIAN_POINT('Origin',(-6.9,2.5,7.8));
#15210=CARTESIAN_POINT('',(-6.9,2.5,7.965));
#15211=CARTESIAN_POINT('Origin',(-6.9,2.5,7.8));
#15212=CARTESIAN_POINT('',(-5.5,2.5,7.965));
#15213=CARTESIAN_POINT('',(-6.9,2.5,7.965));
#15214=CARTESIAN_POINT('Origin',(-5.5,2.5,7.8));
#15215=CARTESIAN_POINT('Origin',(-6.9,2.5,7.8));
#15216=CARTESIAN_POINT('Origin',(-6.9,-2.5,9.2));
#15217=CARTESIAN_POINT('',(-6.9,-2.5,9.365));
#15218=CARTESIAN_POINT('Origin',(-6.9,-2.5,9.2));
#15219=CARTESIAN_POINT('',(-5.5,-2.5,9.365));
#15220=CARTESIAN_POINT('',(-6.9,-2.5,9.365));
#15221=CARTESIAN_POINT('Origin',(-5.5,-2.5,9.2));
#15222=CARTESIAN_POINT('Origin',(-6.9,-2.5,9.2));
#15223=CARTESIAN_POINT('Origin',(-6.9,-2.5,7.8));
#15224=CARTESIAN_POINT('',(-6.9,-2.5,7.965));
#15225=CARTESIAN_POINT('Origin',(-6.9,-2.5,7.8));
#15226=CARTESIAN_POINT('',(-5.5,-2.5,7.965));
#15227=CARTESIAN_POINT('',(-6.9,-2.5,7.965));
#15228=CARTESIAN_POINT('Origin',(-5.5,-2.5,7.8));
#15229=CARTESIAN_POINT('Origin',(-6.9,-2.5,7.8));
#15230=CARTESIAN_POINT('Origin',(-6.9,2.5,9.2));
#15231=CARTESIAN_POINT('',(-6.9,2.5,9.365));
#15232=CARTESIAN_POINT('Origin',(-6.9,2.5,9.2));
#15233=CARTESIAN_POINT('',(-5.5,2.5,9.365));
#15234=CARTESIAN_POINT('',(-6.9,2.5,9.365));
#15235=CARTESIAN_POINT('Origin',(-5.5,2.5,9.2));
#15236=CARTESIAN_POINT('Origin',(-6.9,2.5,9.2));
#15237=CARTESIAN_POINT('Origin',(-6.4,0.,2.7));
#15238=CARTESIAN_POINT('',(-6.4,-2.02066721859313E-17,2.865));
#15239=CARTESIAN_POINT('Origin',(-6.4,0.,2.7));
#15240=CARTESIAN_POINT('',(-5.5,2.02066721859313E-17,2.865));
#15241=CARTESIAN_POINT('',(-6.4,-2.02066721859313E-17,2.865));
#15242=CARTESIAN_POINT('Origin',(-5.5,0.,2.7));
#15243=CARTESIAN_POINT('Origin',(-6.4,0.,2.7));
#15244=CARTESIAN_POINT('Origin',(-6.4,0.,5.3));
#15245=CARTESIAN_POINT('',(-6.4,-2.02066721859313E-17,5.465));
#15246=CARTESIAN_POINT('Origin',(-6.4,0.,5.3));
#15247=CARTESIAN_POINT('',(-5.5,2.02066721859313E-17,5.465));
#15248=CARTESIAN_POINT('',(-6.4,-2.02066721859313E-17,5.465));
#15249=CARTESIAN_POINT('Origin',(-5.5,0.,5.3));
#15250=CARTESIAN_POINT('Origin',(-6.4,0.,5.3));
#15251=CARTESIAN_POINT('Origin',(-8.6,4.2,3.));
#15252=CARTESIAN_POINT('',(-8.5,4.2,3.165));
#15253=CARTESIAN_POINT('Origin',(-8.5,4.2,3.));
#15254=CARTESIAN_POINT('',(-5.5,4.2,3.165));
#15255=CARTESIAN_POINT('',(-8.6,4.2,3.165));
#15256=CARTESIAN_POINT('Origin',(-5.5,4.2,3.));
#15257=CARTESIAN_POINT('Origin',(-8.6,-4.2,5.8));
#15258=CARTESIAN_POINT('',(-8.5,-4.2,5.965));
#15259=CARTESIAN_POINT('Origin',(-8.5,-4.2,5.8));
#15260=CARTESIAN_POINT('',(-5.5,-4.2,5.965));
#15261=CARTESIAN_POINT('',(-8.6,-4.2,5.965));
#15262=CARTESIAN_POINT('Origin',(-5.5,-4.2,5.8));
#15263=CARTESIAN_POINT('Origin',(-8.6,-4.2,3.));
#15264=CARTESIAN_POINT('',(-8.5,-4.2,3.165));
#15265=CARTESIAN_POINT('Origin',(-8.5,-4.2,3.));
#15266=CARTESIAN_POINT('',(-5.5,-4.2,3.165));
#15267=CARTESIAN_POINT('',(-8.6,-4.2,3.165));
#15268=CARTESIAN_POINT('Origin',(-5.5,-4.2,3.));
#15269=CARTESIAN_POINT('Origin',(-8.6,4.2,5.8));
#15270=CARTESIAN_POINT('',(-8.5,4.2,5.965));
#15271=CARTESIAN_POINT('Origin',(-8.5,4.2,5.8));
#15272=CARTESIAN_POINT('',(-5.5,4.2,5.965));
#15273=CARTESIAN_POINT('',(-8.6,4.2,5.965));
#15274=CARTESIAN_POINT('Origin',(-5.5,4.2,5.8));
#15275=CARTESIAN_POINT('Origin',(-8.6,0.,4.));
#15276=CARTESIAN_POINT('',(-8.5,-1.34711147906209E-16,5.1));
#15277=CARTESIAN_POINT('Origin',(-8.5,0.,4.));
#15278=CARTESIAN_POINT('',(-5.5,1.34711147906209E-16,5.1));
#15279=CARTESIAN_POINT('',(-8.6,-1.34711147906209E-16,5.1));
#15280=CARTESIAN_POINT('Origin',(-5.5,0.,4.));
#15281=CARTESIAN_POINT('Origin',(-8.6,-3.,4.));
#15282=CARTESIAN_POINT('',(-8.5,-3.,5.05));
#15283=CARTESIAN_POINT('Origin',(-8.5,-3.,4.));
#15284=CARTESIAN_POINT('',(-5.5,-3.,5.05));
#15285=CARTESIAN_POINT('',(-8.6,-3.,5.05));
#15286=CARTESIAN_POINT('Origin',(-5.5,-3.,4.));
#15287=CARTESIAN_POINT('Origin',(-8.6,3.,4.));
#15288=CARTESIAN_POINT('',(-8.5,3.,5.05));
#15289=CARTESIAN_POINT('Origin',(-8.5,3.,4.));
#15290=CARTESIAN_POINT('',(-5.5,3.,5.05));
#15291=CARTESIAN_POINT('',(-8.6,3.,5.05));
#15292=CARTESIAN_POINT('Origin',(-5.5,3.,4.));
#15293=CARTESIAN_POINT('Origin',(-5.5,4.7,2.3));
#15294=CARTESIAN_POINT('',(-5.5,4.7,2.3));
#15295=CARTESIAN_POINT('',(-8.5,4.7,2.3));
#15296=CARTESIAN_POINT('',(-5.5,4.7,2.3));
#15297=CARTESIAN_POINT('',(-8.5,4.7,10.));
#15298=CARTESIAN_POINT('',(-8.5,4.7,2.3));
#15299=CARTESIAN_POINT('',(-5.5,4.7,10.));
#15300=CARTESIAN_POINT('',(-5.5,4.7,10.));
#15301=CARTESIAN_POINT('',(-5.5,4.7,2.3));
#15302=CARTESIAN_POINT('Origin',(-5.5,-4.7,2.3));
#15303=CARTESIAN_POINT('',(-5.5,-4.7,2.3));
#15304=CARTESIAN_POINT('',(-5.5,-4.7,2.3));
#15305=CARTESIAN_POINT('',(-5.5,-4.7,10.));
#15306=CARTESIAN_POINT('',(-5.5,-4.7,10.));
#15307=CARTESIAN_POINT('',(-5.5,-4.7,2.3));
#15308=CARTESIAN_POINT('Origin',(-8.5,-4.7,2.3));
#15309=CARTESIAN_POINT('',(-8.5,-4.7,2.3));
#15310=CARTESIAN_POINT('',(-8.5,-4.7,2.3));
#15311=CARTESIAN_POINT('',(-8.5,-4.7,10.));
#15312=CARTESIAN_POINT('',(-8.5,-4.7,10.));
#15313=CARTESIAN_POINT('',(-8.5,-4.7,2.3));
#15314=CARTESIAN_POINT('Origin',(-8.5,4.7,2.3));
#15315=CARTESIAN_POINT('',(-8.5,4.7,2.3));
#15316=CARTESIAN_POINT('',(-8.5,4.7,10.));
#15317=CARTESIAN_POINT('Origin',(-7.,0.,10.));
#15318=CARTESIAN_POINT('Origin',(-7.,0.,2.3));
#16725=UNCERTAINTY_MEASURE_WITH_UNIT(LENGTH_MEASURE(0.001),#16800,
'DISTANCE_ACCURACY_VALUE',
'Maximum model space distance between geometric entities at asserted c
onnectivities');
#16750=UNCERTAINTY_MEASURE_WITH_UNIT(LENGTH_MEASURE(0.001),#16800,
'DISTANCE_ACCURACY_VALUE',
'Maximum model space distance between geometric entities at asserted c
onnectivities');
#16774=(
GEOMETRIC_REPRESENTATION_CONTEXT(3)
GLOBAL_UNCERTAINTY_ASSIGNED_CONTEXT((#16725))
GLOBAL_UNIT_ASSIGNED_CONTEXT((#16800,#16802,#16803))
REPRESENTATION_CONTEXT('','3D')
);
#16799=(
GEOMETRIC_REPRESENTATION_CONTEXT(3)
GLOBAL_UNCERTAINTY_ASSIGNED_CONTEXT((#16750))
GLOBAL_UNIT_ASSIGNED_CONTEXT((#16800,#16802,#16803))
REPRESENTATION_CONTEXT('','3D')
);
#16800=(
LENGTH_UNIT()
NAMED_UNIT(*)
SI_UNIT(.CENTI.,.METRE.)
);
#16802=(
NAMED_UNIT(*)
PLANE_ANGLE_UNIT()
SI_UNIT($,.RADIAN.)
);
#16803=(
NAMED_UNIT(*)
SI_UNIT($,.STERADIAN.)
SOLID_ANGLE_UNIT()
);
#16827=SHAPE_DEFINITION_REPRESENTATION(#16880,#17036);
#16880=PRODUCT_DEFINITION_SHAPE('',$,#17085);
#17036=SHAPE_REPRESENTATION('',(#10083),#16774);
#17061=PRODUCT_DEFINITION_CONTEXT('part definition',#17207,'design');
#17085=PRODUCT_DEFINITION('Left jaw body','Left jaw body',#17133,#17061);
#17133=PRODUCT_DEFINITION_FORMATION('',$,#17232);
#17207=APPLICATION_CONTEXT(
'Core Data for Automotive Mechanical Design Process');
#17208=PRODUCT_CONTEXT('part definition',#17207,'mechanical');
#17232=PRODUCT('Left jaw body','Left jaw body','Left jaw body',(#17208));
#17299=COLOUR_RGB('Dark Blue',0.08,0.2,0.34);
#17300=FILL_AREA_STYLE_COLOUR('',#17299);
#17301=FILL_AREA_STYLE('',(#17300));
#17302=SURFACE_STYLE_FILL_AREA(#17301);
#17303=SURFACE_SIDE_STYLE('',(#17302));
#17304=SURFACE_STYLE_USAGE(.BOTH.,#17303);
#17305=PRESENTATION_STYLE_ASSIGNMENT((#17304));
ENDSEC;
END-ISO-10303-21;
